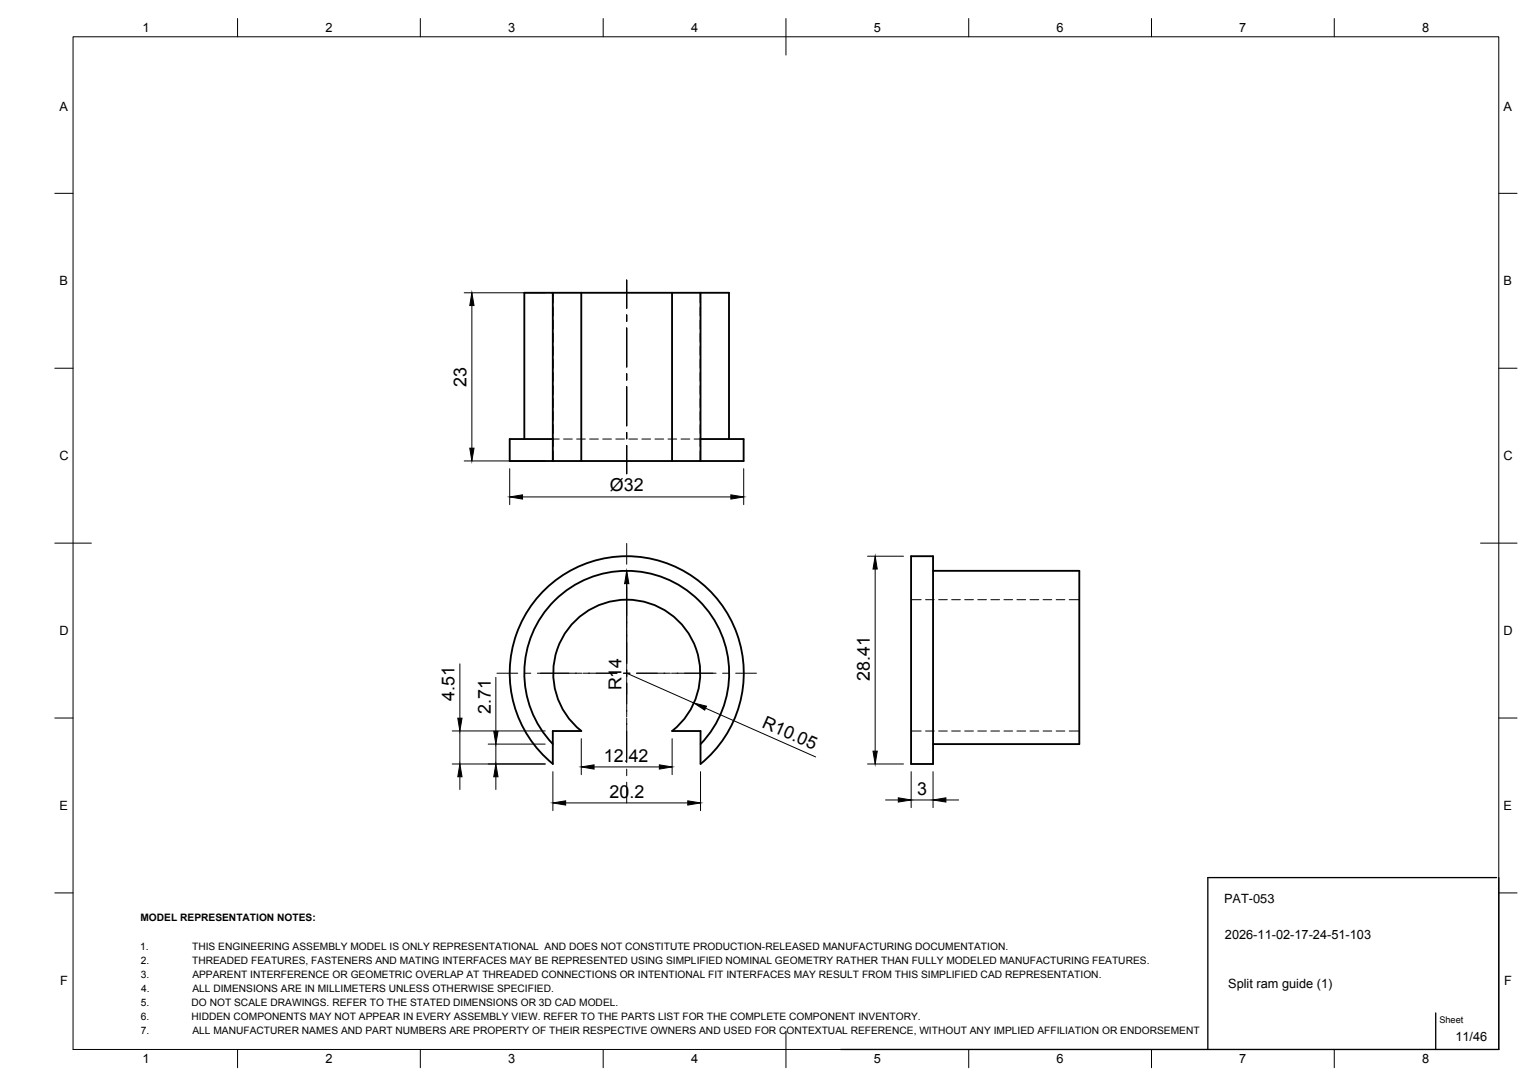
ISO-10303-21;
HEADER;
/* Generated by software containing ST-Developer
 * from STEP Tools, Inc. (www.steptools.com) 
 */

FILE_DESCRIPTION(
/* description */ ('Hand-operated arbor press'),
/* implementation_level */ '2;1');

FILE_NAME(
/* name */ 'Split ram guide (1).step',
/* time_stamp */ '2026-10-28T03:25:25-07:00',
/* author */ (''),
/* organization */ (''),
/* preprocessor_version */ 'ST-DEVELOPER v20.2',
/* originating_system */ 'Autodesk Translation Framework v15.17.0.0',
/* authorisation */ '');

FILE_SCHEMA (('AUTOMOTIVE_DESIGN { 1 0 10303 214 3 1 1 }'));
ENDSEC;

DATA;
#10=MECHANICAL_DESIGN_GEOMETRIC_PRESENTATION_REPRESENTATION('',(#592),#32751);
#508=SHAPE_REPRESENTATION_RELATIONSHIP('SRR','None',#32937,#550);
#550=ADVANCED_BREP_SHAPE_REPRESENTATION('',(#641),#32711);
#592=STYLED_ITEM('',(#33235),#641);
#641=MANIFOLD_SOLID_BREP('Body1',#12489);
#912=PLANE('',#13161);
#913=PLANE('',#13162);
#914=PLANE('',#13163);
#915=PLANE('',#13164);
#916=PLANE('',#13165);
#917=PLANE('',#13172);
#918=PLANE('',#13176);
#1386=FACE_OUTER_BOUND('',#2106,.T.);
#1387=FACE_OUTER_BOUND('',#2107,.T.);
#1388=FACE_OUTER_BOUND('',#2108,.T.);
#1389=FACE_OUTER_BOUND('',#2109,.T.);
#1390=FACE_OUTER_BOUND('',#2110,.T.);
#1391=FACE_OUTER_BOUND('',#2111,.T.);
#1392=FACE_OUTER_BOUND('',#2112,.T.);
#1393=FACE_OUTER_BOUND('',#2113,.T.);
#1394=FACE_OUTER_BOUND('',#2114,.T.);
#1395=FACE_OUTER_BOUND('',#2115,.T.);
#2106=EDGE_LOOP('',(#8768,#8769,#8770,#8771));
#2107=EDGE_LOOP('',(#8772,#8773,#8774,#8775));
#2108=EDGE_LOOP('',(#8776,#8777,#8778,#8779,#8780,#8781));
#2109=EDGE_LOOP('',(#8782,#8783,#8784,#8785,#8786,#8787));
#2110=EDGE_LOOP('',(#8788,#8789,#8790,#8791,#8792,#8793));
#2111=EDGE_LOOP('',(#8794,#8795,#8796,#8797));
#2112=EDGE_LOOP('',(#8798,#8799,#8800,#8801));
#2113=EDGE_LOOP('',(#8802,#8803,#8804,#8805));
#2114=EDGE_LOOP('',(#8806,#8807,#8808,#8809));
#2115=EDGE_LOOP('',(#8810,#8811,#8812,#8813,#8814,#8815));
#2986=LINE('',#18113,#4157);
#2987=LINE('',#18115,#4158);
#2988=LINE('',#18117,#4159);
#2989=LINE('',#18118,#4160);
#2990=LINE('',#18122,#4161);
#2991=LINE('',#18124,#4162);
#2992=LINE('',#18126,#4163);
#2993=LINE('',#18127,#4164);
#2994=LINE('',#18130,#4165);
#2995=LINE('',#18132,#4166);
#2996=LINE('',#18134,#4167);
#2997=LINE('',#18136,#4168);
#2998=LINE('',#18137,#4169);
#2999=LINE('',#18140,#4170);
#3000=LINE('',#18142,#4171);
#3001=LINE('',#18144,#4172);
#3002=LINE('',#18146,#4173);
#3003=LINE('',#18147,#4174);
#4157=VECTOR('',#14643,1.);
#4158=VECTOR('',#14644,1.);
#4159=VECTOR('',#14645,1.);
#4160=VECTOR('',#14646,1.);
#4161=VECTOR('',#14649,1.);
#4162=VECTOR('',#14650,1.);
#4163=VECTOR('',#14651,1.);
#4164=VECTOR('',#14652,1.);
#4165=VECTOR('',#14655,1.);
#4166=VECTOR('',#14656,1.);
#4167=VECTOR('',#14657,1.);
#4168=VECTOR('',#14658,1.);
#4169=VECTOR('',#14659,1.);
#4170=VECTOR('',#14662,1.);
#4171=VECTOR('',#14663,1.);
#4172=VECTOR('',#14664,1.);
#4173=VECTOR('',#14665,1.);
#4174=VECTOR('',#14666,1.);
#5226=CIRCLE('',#13166,1.4);
#5227=CIRCLE('',#13167,1.005);
#5228=CIRCLE('',#13169,1.005);
#5229=CIRCLE('',#13171,1.4);
#5230=CIRCLE('',#13173,1.6);
#5231=CIRCLE('',#13175,1.6);
#5704=VERTEX_POINT('',#18111);
#5705=VERTEX_POINT('',#18112);
#5706=VERTEX_POINT('',#18114);
#5707=VERTEX_POINT('',#18116);
#5708=VERTEX_POINT('',#18120);
#5709=VERTEX_POINT('',#18121);
#5710=VERTEX_POINT('',#18123);
#5711=VERTEX_POINT('',#18125);
#5712=VERTEX_POINT('',#18129);
#5713=VERTEX_POINT('',#18131);
#5714=VERTEX_POINT('',#18133);
#5715=VERTEX_POINT('',#18135);
#5716=VERTEX_POINT('',#18139);
#5717=VERTEX_POINT('',#18141);
#5718=VERTEX_POINT('',#18143);
#5719=VERTEX_POINT('',#18145);
#6887=EDGE_CURVE('',#5704,#5705,#2986,.T.);
#6888=EDGE_CURVE('',#5704,#5706,#2987,.T.);
#6889=EDGE_CURVE('',#5707,#5706,#2988,.T.);
#6890=EDGE_CURVE('',#5705,#5707,#2989,.T.);
#6891=EDGE_CURVE('',#5708,#5709,#2990,.T.);
#6892=EDGE_CURVE('',#5710,#5708,#2991,.T.);
#6893=EDGE_CURVE('',#5711,#5710,#2992,.T.);
#6894=EDGE_CURVE('',#5709,#5711,#2993,.T.);
#6895=EDGE_CURVE('',#5712,#5708,#2994,.T.);
#6896=EDGE_CURVE('',#5713,#5712,#2995,.T.);
#6897=EDGE_CURVE('',#5714,#5713,#2996,.T.);
#6898=EDGE_CURVE('',#5715,#5714,#2997,.T.);
#6899=EDGE_CURVE('',#5710,#5715,#2998,.T.);
#6900=EDGE_CURVE('',#5716,#5704,#2999,.T.);
#6901=EDGE_CURVE('',#5717,#5716,#3000,.T.);
#6902=EDGE_CURVE('',#5718,#5717,#3001,.T.);
#6903=EDGE_CURVE('',#5719,#5718,#3002,.T.);
#6904=EDGE_CURVE('',#5706,#5719,#3003,.T.);
#6905=EDGE_CURVE('',#5716,#5715,#5226,.T.);
#6906=EDGE_CURVE('',#5711,#5705,#5227,.T.);
#6907=EDGE_CURVE('',#5709,#5707,#5228,.T.);
#6908=EDGE_CURVE('',#5717,#5714,#5229,.T.);
#6909=EDGE_CURVE('',#5718,#5713,#5230,.T.);
#6910=EDGE_CURVE('',#5719,#5712,#5231,.T.);
#8768=ORIENTED_EDGE('',*,*,#6887,.F.);
#8769=ORIENTED_EDGE('',*,*,#6888,.T.);
#8770=ORIENTED_EDGE('',*,*,#6889,.F.);
#8771=ORIENTED_EDGE('',*,*,#6890,.F.);
#8772=ORIENTED_EDGE('',*,*,#6891,.F.);
#8773=ORIENTED_EDGE('',*,*,#6892,.F.);
#8774=ORIENTED_EDGE('',*,*,#6893,.F.);
#8775=ORIENTED_EDGE('',*,*,#6894,.F.);
#8776=ORIENTED_EDGE('',*,*,#6895,.F.);
#8777=ORIENTED_EDGE('',*,*,#6896,.F.);
#8778=ORIENTED_EDGE('',*,*,#6897,.F.);
#8779=ORIENTED_EDGE('',*,*,#6898,.F.);
#8780=ORIENTED_EDGE('',*,*,#6899,.F.);
#8781=ORIENTED_EDGE('',*,*,#6892,.T.);
#8782=ORIENTED_EDGE('',*,*,#6900,.F.);
#8783=ORIENTED_EDGE('',*,*,#6901,.F.);
#8784=ORIENTED_EDGE('',*,*,#6902,.F.);
#8785=ORIENTED_EDGE('',*,*,#6903,.F.);
#8786=ORIENTED_EDGE('',*,*,#6904,.F.);
#8787=ORIENTED_EDGE('',*,*,#6888,.F.);
#8788=ORIENTED_EDGE('',*,*,#6893,.T.);
#8789=ORIENTED_EDGE('',*,*,#6899,.T.);
#8790=ORIENTED_EDGE('',*,*,#6905,.F.);
#8791=ORIENTED_EDGE('',*,*,#6900,.T.);
#8792=ORIENTED_EDGE('',*,*,#6887,.T.);
#8793=ORIENTED_EDGE('',*,*,#6906,.F.);
#8794=ORIENTED_EDGE('',*,*,#6894,.T.);
#8795=ORIENTED_EDGE('',*,*,#6906,.T.);
#8796=ORIENTED_EDGE('',*,*,#6890,.T.);
#8797=ORIENTED_EDGE('',*,*,#6907,.F.);
#8798=ORIENTED_EDGE('',*,*,#6898,.T.);
#8799=ORIENTED_EDGE('',*,*,#6908,.F.);
#8800=ORIENTED_EDGE('',*,*,#6901,.T.);
#8801=ORIENTED_EDGE('',*,*,#6905,.T.);
#8802=ORIENTED_EDGE('',*,*,#6897,.T.);
#8803=ORIENTED_EDGE('',*,*,#6909,.F.);
#8804=ORIENTED_EDGE('',*,*,#6902,.T.);
#8805=ORIENTED_EDGE('',*,*,#6908,.T.);
#8806=ORIENTED_EDGE('',*,*,#6896,.T.);
#8807=ORIENTED_EDGE('',*,*,#6910,.F.);
#8808=ORIENTED_EDGE('',*,*,#6903,.T.);
#8809=ORIENTED_EDGE('',*,*,#6909,.T.);
#8810=ORIENTED_EDGE('',*,*,#6891,.T.);
#8811=ORIENTED_EDGE('',*,*,#6907,.T.);
#8812=ORIENTED_EDGE('',*,*,#6889,.T.);
#8813=ORIENTED_EDGE('',*,*,#6904,.T.);
#8814=ORIENTED_EDGE('',*,*,#6910,.T.);
#8815=ORIENTED_EDGE('',*,*,#6895,.T.);
#11672=CYLINDRICAL_SURFACE('',#13168,1.005);
#11673=CYLINDRICAL_SURFACE('',#13170,1.4);
#11674=CYLINDRICAL_SURFACE('',#13174,1.6);
#11895=ADVANCED_FACE('',(#1386),#912,.F.);
#11896=ADVANCED_FACE('',(#1387),#913,.F.);
#11897=ADVANCED_FACE('',(#1388),#914,.F.);
#11898=ADVANCED_FACE('',(#1389),#915,.F.);
#11899=ADVANCED_FACE('',(#1390),#916,.F.);
#11900=ADVANCED_FACE('',(#1391),#11672,.F.);
#11901=ADVANCED_FACE('',(#1392),#11673,.T.);
#11902=ADVANCED_FACE('',(#1393),#917,.F.);
#11903=ADVANCED_FACE('',(#1394),#11674,.T.);
#11904=ADVANCED_FACE('',(#1395),#918,.T.);
#12489=CLOSED_SHELL('',(#11895,#11896,#11897,#11898,#11899,#11900,#11901,
#11902,#11903,#11904));
#13160=AXIS2_PLACEMENT_3D('',#18109,#14639,#14640);
#13161=AXIS2_PLACEMENT_3D('',#18110,#14641,#14642);
#13162=AXIS2_PLACEMENT_3D('',#18119,#14647,#14648);
#13163=AXIS2_PLACEMENT_3D('',#18128,#14653,#14654);
#13164=AXIS2_PLACEMENT_3D('',#18138,#14660,#14661);
#13165=AXIS2_PLACEMENT_3D('',#18148,#14667,#14668);
#13166=AXIS2_PLACEMENT_3D('',#18149,#14669,#14670);
#13167=AXIS2_PLACEMENT_3D('',#18150,#14671,#14672);
#13168=AXIS2_PLACEMENT_3D('',#18151,#14673,#14674);
#13169=AXIS2_PLACEMENT_3D('',#18152,#14675,#14676);
#13170=AXIS2_PLACEMENT_3D('',#18153,#14677,#14678);
#13171=AXIS2_PLACEMENT_3D('',#18154,#14679,#14680);
#13172=AXIS2_PLACEMENT_3D('',#18155,#14681,#14682);
#13173=AXIS2_PLACEMENT_3D('',#18156,#14683,#14684);
#13174=AXIS2_PLACEMENT_3D('',#18157,#14685,#14686);
#13175=AXIS2_PLACEMENT_3D('',#18158,#14687,#14688);
#13176=AXIS2_PLACEMENT_3D('',#18159,#14689,#14690);
#14639=DIRECTION('axis',(0.,0.,1.));
#14640=DIRECTION('refdir',(1.,0.,0.));
#14641=DIRECTION('center_axis',(1.,0.,0.));
#14642=DIRECTION('ref_axis',(0.,1.,0.));
#14643=DIRECTION('',(0.,1.,0.));
#14644=DIRECTION('',(0.,0.,1.));
#14645=DIRECTION('',(0.,-1.,0.));
#14646=DIRECTION('',(0.,0.,1.));
#14647=DIRECTION('center_axis',(1.,0.,0.));
#14648=DIRECTION('ref_axis',(0.,1.,0.));
#14649=DIRECTION('',(0.,-1.,0.));
#14650=DIRECTION('',(0.,0.,1.));
#14651=DIRECTION('',(0.,1.,0.));
#14652=DIRECTION('',(0.,0.,-1.));
#14653=DIRECTION('center_axis',(0.,1.,0.));
#14654=DIRECTION('ref_axis',(-1.,0.,0.));
#14655=DIRECTION('',(1.,0.,0.));
#14656=DIRECTION('',(0.,0.,1.));
#14657=DIRECTION('',(-1.,0.,0.));
#14658=DIRECTION('',(0.,0.,1.));
#14659=DIRECTION('',(-1.,0.,0.));
#14660=DIRECTION('center_axis',(0.,-1.,0.));
#14661=DIRECTION('ref_axis',(1.,0.,0.));
#14662=DIRECTION('',(1.,0.,0.));
#14663=DIRECTION('',(0.,0.,-1.));
#14664=DIRECTION('',(1.,0.,0.));
#14665=DIRECTION('',(0.,0.,-1.));
#14666=DIRECTION('',(-1.,0.,0.));
#14667=DIRECTION('center_axis',(0.,0.,1.));
#14668=DIRECTION('ref_axis',(1.,0.,0.));
#14669=DIRECTION('center_axis',(0.,0.,1.));
#14670=DIRECTION('ref_axis',(1.,0.,0.));
#14671=DIRECTION('center_axis',(0.,0.,-1.));
#14672=DIRECTION('ref_axis',(1.,0.,0.));
#14673=DIRECTION('center_axis',(0.,0.,1.));
#14674=DIRECTION('ref_axis',(1.,0.,0.));
#14675=DIRECTION('center_axis',(0.,0.,-1.));
#14676=DIRECTION('ref_axis',(1.,0.,0.));
#14677=DIRECTION('center_axis',(0.,0.,1.));
#14678=DIRECTION('ref_axis',(1.,0.,0.));
#14679=DIRECTION('center_axis',(0.,0.,1.));
#14680=DIRECTION('ref_axis',(1.,0.,0.));
#14681=DIRECTION('center_axis',(0.,0.,1.));
#14682=DIRECTION('ref_axis',(1.,0.,0.));
#14683=DIRECTION('center_axis',(0.,0.,1.));
#14684=DIRECTION('ref_axis',(1.,0.,0.));
#14685=DIRECTION('center_axis',(0.,0.,1.));
#14686=DIRECTION('ref_axis',(1.,0.,0.));
#14687=DIRECTION('center_axis',(0.,0.,1.));
#14688=DIRECTION('ref_axis',(1.,0.,0.));
#14689=DIRECTION('center_axis',(0.,0.,1.));
#14690=DIRECTION('ref_axis',(1.,0.,0.));
#18109=CARTESIAN_POINT('',(0.,0.,0.));
#18110=CARTESIAN_POINT('Origin',(0.21,-1.01,22.9));
#18111=CARTESIAN_POINT('',(0.21,-1.01,23.));
#18112=CARTESIAN_POINT('',(0.21,-0.621228621362538,23.));
#18113=CARTESIAN_POINT('',(0.21,-0.505,23.));
#18114=CARTESIAN_POINT('',(0.21,-1.01,25.3));
#18115=CARTESIAN_POINT('',(0.21,-1.01,22.9));
#18116=CARTESIAN_POINT('',(0.21,-0.621228621362538,25.3));
#18117=CARTESIAN_POINT('',(0.21,-0.505,25.3));
#18118=CARTESIAN_POINT('',(0.21,-0.621228621362538,23.));
#18119=CARTESIAN_POINT('Origin',(0.21,-1.01,22.9));
#18120=CARTESIAN_POINT('',(0.21,1.01,25.3));
#18121=CARTESIAN_POINT('',(0.21,0.621228621362538,25.3));
#18122=CARTESIAN_POINT('',(0.21,-0.505,25.3));
#18123=CARTESIAN_POINT('',(0.21,1.01,23.));
#18124=CARTESIAN_POINT('',(0.21,1.01,22.9));
#18125=CARTESIAN_POINT('',(0.21,0.621228621362538,23.));
#18126=CARTESIAN_POINT('',(0.21,-0.505,23.));
#18127=CARTESIAN_POINT('',(0.21,0.621228621362538,23.));
#18128=CARTESIAN_POINT('Origin',(0.21,1.01,22.9));
#18129=CARTESIAN_POINT('',(-0.240927072796786,1.01,25.3));
#18130=CARTESIAN_POINT('',(0.605,1.01,25.3));
#18131=CARTESIAN_POINT('',(-0.240927072796786,1.01,25.));
#18132=CARTESIAN_POINT('',(-0.240927072796786,1.01,25.));
#18133=CARTESIAN_POINT('',(0.0305156009506911,1.01,25.));
#18134=CARTESIAN_POINT('',(0.605,1.01,25.));
#18135=CARTESIAN_POINT('',(0.0305156009506911,1.01,23.));
#18136=CARTESIAN_POINT('',(0.0305156009506911,1.01,23.));
#18137=CARTESIAN_POINT('',(0.605,1.01,23.));
#18138=CARTESIAN_POINT('Origin',(-0.7,-1.01,22.9));
#18139=CARTESIAN_POINT('',(0.0305156009506911,-1.01,23.));
#18140=CARTESIAN_POINT('',(0.15,-1.01,23.));
#18141=CARTESIAN_POINT('',(0.0305156009506911,-1.01,25.));
#18142=CARTESIAN_POINT('',(0.0305156009506911,-1.01,23.));
#18143=CARTESIAN_POINT('',(-0.240927072796786,-1.01,25.));
#18144=CARTESIAN_POINT('',(0.15,-1.01,25.));
#18145=CARTESIAN_POINT('',(-0.240927072796786,-1.01,25.3));
#18146=CARTESIAN_POINT('',(-0.240927072796786,-1.01,25.));
#18147=CARTESIAN_POINT('',(0.15,-1.01,25.3));
#18148=CARTESIAN_POINT('Origin',(1.,0.,23.));
#18149=CARTESIAN_POINT('Origin',(1.,0.,23.));
#18150=CARTESIAN_POINT('Origin',(1.,0.,23.));
#18151=CARTESIAN_POINT('Origin',(1.,0.,23.));
#18152=CARTESIAN_POINT('Origin',(1.,0.,25.3));
#18153=CARTESIAN_POINT('Origin',(1.,0.,23.));
#18154=CARTESIAN_POINT('Origin',(1.,0.,25.));
#18155=CARTESIAN_POINT('Origin',(1.,0.,25.));
#18156=CARTESIAN_POINT('Origin',(1.,0.,25.));
#18157=CARTESIAN_POINT('Origin',(1.,0.,25.));
#18158=CARTESIAN_POINT('Origin',(1.,0.,25.3));
#18159=CARTESIAN_POINT('Origin',(1.,0.,25.3));
#32662=UNCERTAINTY_MEASURE_WITH_UNIT(LENGTH_MEASURE(0.001),#32752,
'DISTANCE_ACCURACY_VALUE',
'Maximum model space distance between geometric entities at asserted c
onnectivities');
#32702=UNCERTAINTY_MEASURE_WITH_UNIT(LENGTH_MEASURE(0.001),#32752,
'DISTANCE_ACCURACY_VALUE',
'Maximum model space distance between geometric entities at asserted c
onnectivities');
#32711=(
GEOMETRIC_REPRESENTATION_CONTEXT(3)
GLOBAL_UNCERTAINTY_ASSIGNED_CONTEXT((#32662))
GLOBAL_UNIT_ASSIGNED_CONTEXT((#32752,#32754,#32755))
REPRESENTATION_CONTEXT('','3D')
);
#32751=(
GEOMETRIC_REPRESENTATION_CONTEXT(3)
GLOBAL_UNCERTAINTY_ASSIGNED_CONTEXT((#32702))
GLOBAL_UNIT_ASSIGNED_CONTEXT((#32752,#32754,#32755))
REPRESENTATION_CONTEXT('','3D')
);
#32752=(
LENGTH_UNIT()
NAMED_UNIT(*)
SI_UNIT(.CENTI.,.METRE.)
);
#32754=(
NAMED_UNIT(*)
PLANE_ANGLE_UNIT()
SI_UNIT($,.RADIAN.)
);
#32755=(
NAMED_UNIT(*)
SI_UNIT($,.STERADIAN.)
SOLID_ANGLE_UNIT()
);
#32764=SHAPE_DEFINITION_REPRESENTATION(#32812,#32937);
#32812=PRODUCT_DEFINITION_SHAPE('',$,#32986);
#32937=SHAPE_REPRESENTATION('',(#13160),#32711);
#32977=PRODUCT_DEFINITION_CONTEXT('part definition',#33123,'design');
#32986=PRODUCT_DEFINITION('Split ram guide (1)','Split ram guide (1)',#33034,
#32977);
#33034=PRODUCT_DEFINITION_FORMATION('',$,#33133);
#33123=APPLICATION_CONTEXT(
'Core Data for Automotive Mechanical Design Process');
#33124=PRODUCT_CONTEXT('part definition',#33123,'mechanical');
#33133=PRODUCT('Split ram guide (1)','Split ram guide (1)',
'Split ram guide (1)',(#33124));
#33229=COLOUR_RGB('Sky Blue',0.24,0.69,0.87);
#33230=FILL_AREA_STYLE_COLOUR('',#33229);
#33231=FILL_AREA_STYLE('',(#33230));
#33232=SURFACE_STYLE_FILL_AREA(#33231);
#33233=SURFACE_SIDE_STYLE('',(#33232));
#33234=SURFACE_STYLE_USAGE(.BOTH.,#33233);
#33235=PRESENTATION_STYLE_ASSIGNMENT((#33234));
ENDSEC;
END-ISO-10303-21;
